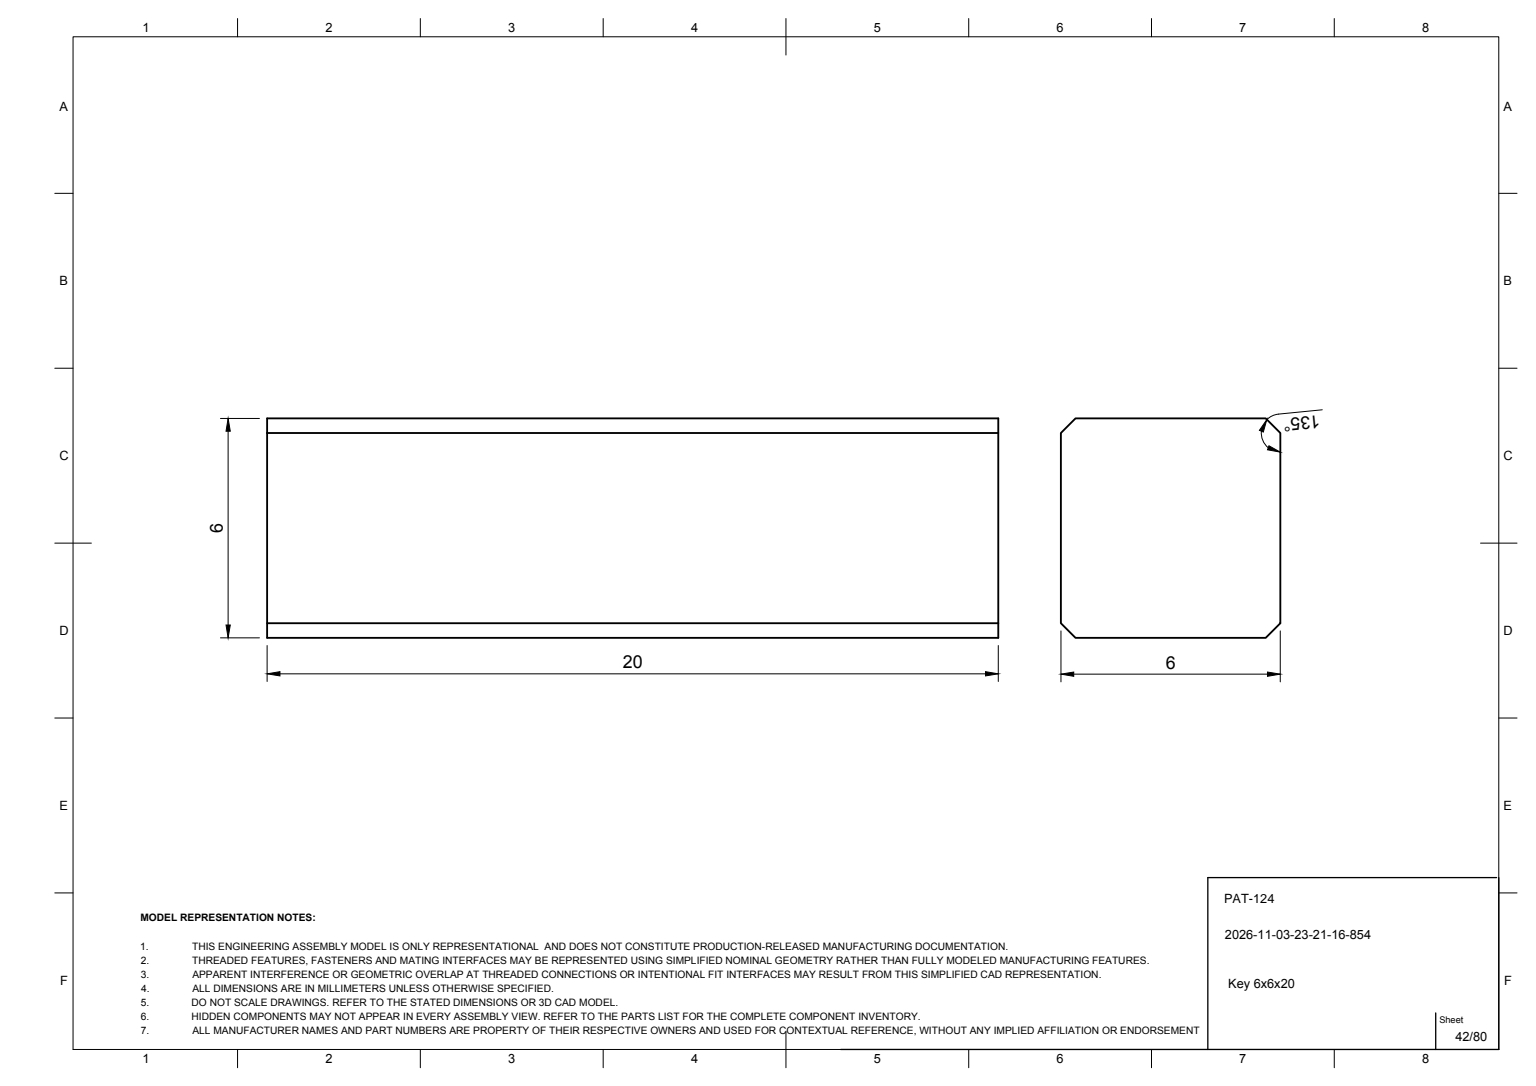
ISO-10303-21;
HEADER;
/* Generated by software containing ST-Developer
 * from STEP Tools, Inc. (www.steptools.com) 
 */

FILE_DESCRIPTION(
/* description */ ('XY cross-slide table'),
/* implementation_level */ '2;1');

FILE_NAME(
/* name */ 'Key 6x6x20.step',
/* time_stamp */ '2026-10-28T03:22:46-07:00',
/* author */ (''),
/* organization */ (''),
/* preprocessor_version */ 'ST-DEVELOPER v20.2',
/* originating_system */ 'Autodesk Translation Framework v15.17.0.0',
/* authorisation */ '');

FILE_SCHEMA (('AUTOMOTIVE_DESIGN { 1 0 10303 214 3 1 1 }'));
ENDSEC;

DATA;
#10=MECHANICAL_DESIGN_GEOMETRIC_PRESENTATION_REPRESENTATION('',(#1723),#62984);
#1542=SHAPE_REPRESENTATION_RELATIONSHIP('SRR','None',#63395,#1625);
#1625=ADVANCED_BREP_SHAPE_REPRESENTATION('',(#1833),#62932);
#1723=STYLED_ITEM('',(#63912),#1833);
#1833=MANIFOLD_SOLID_BREP('Body1',#23020);
#2545=PLANE('',#25091);
#2546=PLANE('',#25092);
#2547=PLANE('',#25093);
#2548=PLANE('',#25094);
#2549=PLANE('',#25095);
#2550=PLANE('',#25096);
#2551=PLANE('',#25097);
#2552=PLANE('',#25098);
#2553=PLANE('',#25099);
#2554=PLANE('',#25100);
#3469=FACE_OUTER_BOUND('',#4977,.T.);
#3470=FACE_OUTER_BOUND('',#4978,.T.);
#3471=FACE_OUTER_BOUND('',#4979,.T.);
#3472=FACE_OUTER_BOUND('',#4980,.T.);
#3473=FACE_OUTER_BOUND('',#4981,.T.);
#3474=FACE_OUTER_BOUND('',#4982,.T.);
#3475=FACE_OUTER_BOUND('',#4983,.T.);
#3476=FACE_OUTER_BOUND('',#4984,.T.);
#3477=FACE_OUTER_BOUND('',#4985,.T.);
#3478=FACE_OUTER_BOUND('',#4986,.T.);
#4977=EDGE_LOOP('',(#17756,#17757,#17758,#17759,#17760,#17761,#17762,#17763));
#4978=EDGE_LOOP('',(#17764,#17765,#17766,#17767));
#4979=EDGE_LOOP('',(#17768,#17769,#17770,#17771));
#4980=EDGE_LOOP('',(#17772,#17773,#17774,#17775));
#4981=EDGE_LOOP('',(#17776,#17777,#17778,#17779));
#4982=EDGE_LOOP('',(#17780,#17781,#17782,#17783,#17784,#17785,#17786,#17787));
#4983=EDGE_LOOP('',(#17788,#17789,#17790,#17791));
#4984=EDGE_LOOP('',(#17792,#17793,#17794,#17795));
#4985=EDGE_LOOP('',(#17796,#17797,#17798,#17799));
#4986=EDGE_LOOP('',(#17800,#17801,#17802,#17803));
#6573=LINE('',#47546,#8060);
#6574=LINE('',#47548,#8061);
#6575=LINE('',#47550,#8062);
#6576=LINE('',#47552,#8063);
#6577=LINE('',#47554,#8064);
#6578=LINE('',#47556,#8065);
#6579=LINE('',#47558,#8066);
#6580=LINE('',#47559,#8067);
#6581=LINE('',#47562,#8068);
#6582=LINE('',#47564,#8069);
#6583=LINE('',#47565,#8070);
#6584=LINE('',#47568,#8071);
#6585=LINE('',#47569,#8072);
#6586=LINE('',#47572,#8073);
#6587=LINE('',#47573,#8074);
#6588=LINE('',#47576,#8075);
#6589=LINE('',#47577,#8076);
#6590=LINE('',#47581,#8077);
#6591=LINE('',#47582,#8078);
#6592=LINE('',#47584,#8079);
#6593=LINE('',#47585,#8080);
#6594=LINE('',#47587,#8081);
#6595=LINE('',#47589,#8082);
#6596=LINE('',#47591,#8083);
#8060=VECTOR('',#29312,1.);
#8061=VECTOR('',#29313,1.);
#8062=VECTOR('',#29314,1.);
#8063=VECTOR('',#29315,1.);
#8064=VECTOR('',#29316,1.);
#8065=VECTOR('',#29317,1.);
#8066=VECTOR('',#29318,1.);
#8067=VECTOR('',#29319,1.);
#8068=VECTOR('',#29322,1.);
#8069=VECTOR('',#29323,1.);
#8070=VECTOR('',#29324,1.);
#8071=VECTOR('',#29327,1.);
#8072=VECTOR('',#29328,1.);
#8073=VECTOR('',#29331,1.);
#8074=VECTOR('',#29332,1.);
#8075=VECTOR('',#29335,1.);
#8076=VECTOR('',#29336,1.);
#8077=VECTOR('',#29339,1.);
#8078=VECTOR('',#29340,1.);
#8079=VECTOR('',#29341,1.);
#8080=VECTOR('',#29342,1.);
#8081=VECTOR('',#29345,1.);
#8082=VECTOR('',#29348,1.);
#8083=VECTOR('',#29351,1.);
#10735=VERTEX_POINT('',#47544);
#10736=VERTEX_POINT('',#47545);
#10737=VERTEX_POINT('',#47547);
#10738=VERTEX_POINT('',#47549);
#10739=VERTEX_POINT('',#47551);
#10740=VERTEX_POINT('',#47553);
#10741=VERTEX_POINT('',#47555);
#10742=VERTEX_POINT('',#47557);
#10743=VERTEX_POINT('',#47561);
#10744=VERTEX_POINT('',#47563);
#10745=VERTEX_POINT('',#47567);
#10746=VERTEX_POINT('',#47571);
#10747=VERTEX_POINT('',#47575);
#10748=VERTEX_POINT('',#47579);
#10749=VERTEX_POINT('',#47580);
#10750=VERTEX_POINT('',#47583);
#13262=EDGE_CURVE('',#10735,#10736,#6573,.T.);
#13263=EDGE_CURVE('',#10737,#10735,#6574,.T.);
#13264=EDGE_CURVE('',#10738,#10737,#6575,.T.);
#13265=EDGE_CURVE('',#10739,#10738,#6576,.T.);
#13266=EDGE_CURVE('',#10740,#10739,#6577,.T.);
#13267=EDGE_CURVE('',#10741,#10740,#6578,.T.);
#13268=EDGE_CURVE('',#10742,#10741,#6579,.T.);
#13269=EDGE_CURVE('',#10736,#10742,#6580,.T.);
#13270=EDGE_CURVE('',#10739,#10743,#6581,.T.);
#13271=EDGE_CURVE('',#10743,#10744,#6582,.T.);
#13272=EDGE_CURVE('',#10744,#10740,#6583,.T.);
#13273=EDGE_CURVE('',#10745,#10738,#6584,.T.);
#13274=EDGE_CURVE('',#10745,#10743,#6585,.T.);
#13275=EDGE_CURVE('',#10737,#10746,#6586,.T.);
#13276=EDGE_CURVE('',#10746,#10745,#6587,.T.);
#13277=EDGE_CURVE('',#10747,#10735,#6588,.T.);
#13278=EDGE_CURVE('',#10747,#10746,#6589,.T.);
#13279=EDGE_CURVE('',#10748,#10749,#6590,.T.);
#13280=EDGE_CURVE('',#10744,#10748,#6591,.T.);
#13281=EDGE_CURVE('',#10750,#10747,#6592,.T.);
#13282=EDGE_CURVE('',#10749,#10750,#6593,.T.);
#13283=EDGE_CURVE('',#10741,#10748,#6594,.T.);
#13284=EDGE_CURVE('',#10736,#10750,#6595,.T.);
#13285=EDGE_CURVE('',#10749,#10742,#6596,.T.);
#17756=ORIENTED_EDGE('',*,*,#13262,.F.);
#17757=ORIENTED_EDGE('',*,*,#13263,.F.);
#17758=ORIENTED_EDGE('',*,*,#13264,.F.);
#17759=ORIENTED_EDGE('',*,*,#13265,.F.);
#17760=ORIENTED_EDGE('',*,*,#13266,.F.);
#17761=ORIENTED_EDGE('',*,*,#13267,.F.);
#17762=ORIENTED_EDGE('',*,*,#13268,.F.);
#17763=ORIENTED_EDGE('',*,*,#13269,.F.);
#17764=ORIENTED_EDGE('',*,*,#13266,.T.);
#17765=ORIENTED_EDGE('',*,*,#13270,.T.);
#17766=ORIENTED_EDGE('',*,*,#13271,.T.);
#17767=ORIENTED_EDGE('',*,*,#13272,.T.);
#17768=ORIENTED_EDGE('',*,*,#13265,.T.);
#17769=ORIENTED_EDGE('',*,*,#13273,.F.);
#17770=ORIENTED_EDGE('',*,*,#13274,.T.);
#17771=ORIENTED_EDGE('',*,*,#13270,.F.);
#17772=ORIENTED_EDGE('',*,*,#13264,.T.);
#17773=ORIENTED_EDGE('',*,*,#13275,.T.);
#17774=ORIENTED_EDGE('',*,*,#13276,.T.);
#17775=ORIENTED_EDGE('',*,*,#13273,.T.);
#17776=ORIENTED_EDGE('',*,*,#13263,.T.);
#17777=ORIENTED_EDGE('',*,*,#13277,.F.);
#17778=ORIENTED_EDGE('',*,*,#13278,.T.);
#17779=ORIENTED_EDGE('',*,*,#13275,.F.);
#17780=ORIENTED_EDGE('',*,*,#13279,.F.);
#17781=ORIENTED_EDGE('',*,*,#13280,.F.);
#17782=ORIENTED_EDGE('',*,*,#13271,.F.);
#17783=ORIENTED_EDGE('',*,*,#13274,.F.);
#17784=ORIENTED_EDGE('',*,*,#13276,.F.);
#17785=ORIENTED_EDGE('',*,*,#13278,.F.);
#17786=ORIENTED_EDGE('',*,*,#13281,.F.);
#17787=ORIENTED_EDGE('',*,*,#13282,.F.);
#17788=ORIENTED_EDGE('',*,*,#13267,.T.);
#17789=ORIENTED_EDGE('',*,*,#13272,.F.);
#17790=ORIENTED_EDGE('',*,*,#13280,.T.);
#17791=ORIENTED_EDGE('',*,*,#13283,.F.);
#17792=ORIENTED_EDGE('',*,*,#13262,.T.);
#17793=ORIENTED_EDGE('',*,*,#13284,.T.);
#17794=ORIENTED_EDGE('',*,*,#13281,.T.);
#17795=ORIENTED_EDGE('',*,*,#13277,.T.);
#17796=ORIENTED_EDGE('',*,*,#13268,.T.);
#17797=ORIENTED_EDGE('',*,*,#13283,.T.);
#17798=ORIENTED_EDGE('',*,*,#13279,.T.);
#17799=ORIENTED_EDGE('',*,*,#13285,.T.);
#17800=ORIENTED_EDGE('',*,*,#13269,.T.);
#17801=ORIENTED_EDGE('',*,*,#13285,.F.);
#17802=ORIENTED_EDGE('',*,*,#13282,.T.);
#17803=ORIENTED_EDGE('',*,*,#13284,.F.);
#22250=ADVANCED_FACE('',(#3469),#2545,.F.);
#22251=ADVANCED_FACE('',(#3470),#2546,.T.);
#22252=ADVANCED_FACE('',(#3471),#2547,.T.);
#22253=ADVANCED_FACE('',(#3472),#2548,.T.);
#22254=ADVANCED_FACE('',(#3473),#2549,.T.);
#22255=ADVANCED_FACE('',(#3474),#2550,.T.);
#22256=ADVANCED_FACE('',(#3475),#2551,.F.);
#22257=ADVANCED_FACE('',(#3476),#2552,.T.);
#22258=ADVANCED_FACE('',(#3477),#2553,.T.);
#22259=ADVANCED_FACE('',(#3478),#2554,.T.);
#23020=CLOSED_SHELL('',(#22250,#22251,#22252,#22253,#22254,#22255,#22256,
#22257,#22258,#22259));
#25090=AXIS2_PLACEMENT_3D('',#47542,#29308,#29309);
#25091=AXIS2_PLACEMENT_3D('',#47543,#29310,#29311);
#25092=AXIS2_PLACEMENT_3D('',#47560,#29320,#29321);
#25093=AXIS2_PLACEMENT_3D('',#47566,#29325,#29326);
#25094=AXIS2_PLACEMENT_3D('',#47570,#29329,#29330);
#25095=AXIS2_PLACEMENT_3D('',#47574,#29333,#29334);
#25096=AXIS2_PLACEMENT_3D('',#47578,#29337,#29338);
#25097=AXIS2_PLACEMENT_3D('',#47586,#29343,#29344);
#25098=AXIS2_PLACEMENT_3D('',#47588,#29346,#29347);
#25099=AXIS2_PLACEMENT_3D('',#47590,#29349,#29350);
#25100=AXIS2_PLACEMENT_3D('',#47592,#29352,#29353);
#29308=DIRECTION('axis',(0.,0.,1.));
#29309=DIRECTION('refdir',(1.,0.,0.));
#29310=DIRECTION('center_axis',(1.,0.,0.));
#29311=DIRECTION('ref_axis',(0.,0.,-1.));
#29312=DIRECTION('',(0.,-0.707106781186547,-0.707106781186548));
#29313=DIRECTION('',(0.,-1.,0.));
#29314=DIRECTION('',(0.,-0.707106781186547,0.707106781186548));
#29315=DIRECTION('',(0.,0.,1.));
#29316=DIRECTION('',(0.,0.707106781186547,0.707106781186548));
#29317=DIRECTION('',(0.,1.,0.));
#29318=DIRECTION('',(0.,0.707106781186547,-0.707106781186548));
#29319=DIRECTION('',(0.,0.,-1.));
#29320=DIRECTION('center_axis',(0.,0.707106781186548,-0.707106781186547));
#29321=DIRECTION('ref_axis',(-1.,0.,0.));
#29322=DIRECTION('',(1.,0.,0.));
#29323=DIRECTION('',(0.,-0.707106781186547,-0.707106781186548));
#29324=DIRECTION('',(-1.,0.,0.));
#29325=DIRECTION('center_axis',(0.,1.,0.));
#29326=DIRECTION('ref_axis',(-1.,0.,0.));
#29327=DIRECTION('',(-1.,0.,0.));
#29328=DIRECTION('',(0.,0.,-1.));
#29329=DIRECTION('center_axis',(0.,0.707106781186548,0.707106781186547));
#29330=DIRECTION('ref_axis',(1.,0.,0.));
#29331=DIRECTION('',(1.,0.,0.));
#29332=DIRECTION('',(0.,0.707106781186547,-0.707106781186548));
#29333=DIRECTION('center_axis',(0.,0.,1.));
#29334=DIRECTION('ref_axis',(1.,0.,0.));
#29335=DIRECTION('',(-1.,0.,0.));
#29336=DIRECTION('',(0.,1.,0.));
#29337=DIRECTION('center_axis',(1.,0.,0.));
#29338=DIRECTION('ref_axis',(0.,0.,-1.));
#29339=DIRECTION('',(0.,-0.707106781186547,0.707106781186548));
#29340=DIRECTION('',(0.,-1.,0.));
#29341=DIRECTION('',(0.,0.707106781186547,0.707106781186548));
#29342=DIRECTION('',(0.,0.,1.));
#29343=DIRECTION('center_axis',(0.,0.,1.));
#29344=DIRECTION('ref_axis',(1.,0.,0.));
#29345=DIRECTION('',(1.,0.,0.));
#29346=DIRECTION('center_axis',(0.,-0.707106781186548,0.707106781186547));
#29347=DIRECTION('ref_axis',(1.,0.,0.));
#29348=DIRECTION('',(1.,0.,0.));
#29349=DIRECTION('center_axis',(0.,-0.707106781186548,-0.707106781186547));
#29350=DIRECTION('ref_axis',(-1.,0.,0.));
#29351=DIRECTION('',(-1.,0.,0.));
#29352=DIRECTION('center_axis',(0.,-1.,0.));
#29353=DIRECTION('ref_axis',(1.,0.,0.));
#47542=CARTESIAN_POINT('',(0.,0.,0.));
#47543=CARTESIAN_POINT('Origin',(-1.,0.,0.35));
#47544=CARTESIAN_POINT('',(-1.,-0.26,0.6));
#47545=CARTESIAN_POINT('',(-1.,-0.3,0.56));
#47546=CARTESIAN_POINT('',(-1.,-0.2675,0.5925));
#47547=CARTESIAN_POINT('',(-1.,0.26,0.6));
#47548=CARTESIAN_POINT('',(-1.,0.,0.6));
#47549=CARTESIAN_POINT('',(-1.,0.3,0.56));
#47550=CARTESIAN_POINT('',(-1.,0.2675,0.5925));
#47551=CARTESIAN_POINT('',(-1.,0.3,0.04));
#47552=CARTESIAN_POINT('',(-1.,0.3,0.175));
#47553=CARTESIAN_POINT('',(-1.,0.26,0.));
#47554=CARTESIAN_POINT('',(-1.,0.2925,0.0325));
#47555=CARTESIAN_POINT('',(-1.,-0.26,0.));
#47556=CARTESIAN_POINT('',(-1.,0.,0.));
#47557=CARTESIAN_POINT('',(-1.,-0.3,0.04));
#47558=CARTESIAN_POINT('',(-1.,-0.2925,0.0325));
#47559=CARTESIAN_POINT('',(-1.,-0.3,0.175));
#47560=CARTESIAN_POINT('Origin',(0.75,0.28,0.02));
#47561=CARTESIAN_POINT('',(1.,0.3,0.04));
#47562=CARTESIAN_POINT('',(0.75,0.3,0.04));
#47563=CARTESIAN_POINT('',(1.,0.26,0.));
#47564=CARTESIAN_POINT('',(1.,0.2925,0.0325));
#47565=CARTESIAN_POINT('',(0.75,0.26,0.));
#47566=CARTESIAN_POINT('Origin',(1.5,0.3,0.));
#47567=CARTESIAN_POINT('',(1.,0.3,0.56));
#47568=CARTESIAN_POINT('',(0.75,0.3,0.56));
#47569=CARTESIAN_POINT('',(1.,0.3,0.175));
#47570=CARTESIAN_POINT('Origin',(0.75,0.28,0.58));
#47571=CARTESIAN_POINT('',(1.,0.26,0.6));
#47572=CARTESIAN_POINT('',(0.75,0.26,0.6));
#47573=CARTESIAN_POINT('',(1.,0.2675,0.5925));
#47574=CARTESIAN_POINT('Origin',(0.,0.,0.6));
#47575=CARTESIAN_POINT('',(1.,-0.26,0.6));
#47576=CARTESIAN_POINT('',(-0.75,-0.26,0.6));
#47577=CARTESIAN_POINT('',(1.,0.,0.6));
#47578=CARTESIAN_POINT('Origin',(1.,0.,0.35));
#47579=CARTESIAN_POINT('',(1.,-0.26,0.));
#47580=CARTESIAN_POINT('',(1.,-0.3,0.04));
#47581=CARTESIAN_POINT('',(1.,-0.2925,0.0325));
#47582=CARTESIAN_POINT('',(1.,0.,0.));
#47583=CARTESIAN_POINT('',(1.,-0.3,0.56));
#47584=CARTESIAN_POINT('',(1.,-0.2675,0.5925));
#47585=CARTESIAN_POINT('',(1.,-0.3,0.175));
#47586=CARTESIAN_POINT('Origin',(0.,0.,0.));
#47587=CARTESIAN_POINT('',(-0.75,-0.26,0.));
#47588=CARTESIAN_POINT('Origin',(-0.75,-0.28,0.58));
#47589=CARTESIAN_POINT('',(-0.75,-0.3,0.56));
#47590=CARTESIAN_POINT('Origin',(-0.75,-0.28,0.02));
#47591=CARTESIAN_POINT('',(-0.75,-0.3,0.04));
#47592=CARTESIAN_POINT('Origin',(-1.5,-0.3,0.));
#62833=UNCERTAINTY_MEASURE_WITH_UNIT(LENGTH_MEASURE(0.001),#62985,
'DISTANCE_ACCURACY_VALUE',
'Maximum model space distance between geometric entities at asserted c
onnectivities');
#62885=UNCERTAINTY_MEASURE_WITH_UNIT(LENGTH_MEASURE(0.001),#62985,
'DISTANCE_ACCURACY_VALUE',
'Maximum model space distance between geometric entities at asserted c
onnectivities');
#62932=(
GEOMETRIC_REPRESENTATION_CONTEXT(3)
GLOBAL_UNCERTAINTY_ASSIGNED_CONTEXT((#62833))
GLOBAL_UNIT_ASSIGNED_CONTEXT((#62985,#62987,#62988))
REPRESENTATION_CONTEXT('','3D')
);
#62984=(
GEOMETRIC_REPRESENTATION_CONTEXT(3)
GLOBAL_UNCERTAINTY_ASSIGNED_CONTEXT((#62885))
GLOBAL_UNIT_ASSIGNED_CONTEXT((#62985,#62987,#62988))
REPRESENTATION_CONTEXT('','3D')
);
#62985=(
LENGTH_UNIT()
NAMED_UNIT(*)
SI_UNIT(.CENTI.,.METRE.)
);
#62987=(
NAMED_UNIT(*)
PLANE_ANGLE_UNIT()
SI_UNIT($,.RADIAN.)
);
#62988=(
NAMED_UNIT(*)
SI_UNIT($,.STERADIAN.)
SOLID_ANGLE_UNIT()
);
#63035=SHAPE_DEFINITION_REPRESENTATION(#63166,#63395);
#63166=PRODUCT_DEFINITION_SHAPE('',$,#63494);
#63395=SHAPE_REPRESENTATION('',(#25090),#62932);
#63447=PRODUCT_DEFINITION_CONTEXT('part definition',#63743,'design');
#63494=PRODUCT_DEFINITION('Key 6x6x20','Key 6x6x20',#63592,#63447);
#63592=PRODUCT_DEFINITION_FORMATION('',$,#63791);
#63743=APPLICATION_CONTEXT(
'Core Data for Automotive Mechanical Design Process');
#63744=PRODUCT_CONTEXT('part definition',#63743,'mechanical');
#63791=PRODUCT('Key 6x6x20','Key 6x6x20','Key 6x6x20',(#63744));
#63906=COLOUR_RGB('Grey',0.48,0.52,0.57);
#63907=FILL_AREA_STYLE_COLOUR('',#63906);
#63908=FILL_AREA_STYLE('',(#63907));
#63909=SURFACE_STYLE_FILL_AREA(#63908);
#63910=SURFACE_SIDE_STYLE('',(#63909));
#63911=SURFACE_STYLE_USAGE(.BOTH.,#63910);
#63912=PRESENTATION_STYLE_ASSIGNMENT((#63911));
ENDSEC;
END-ISO-10303-21;
